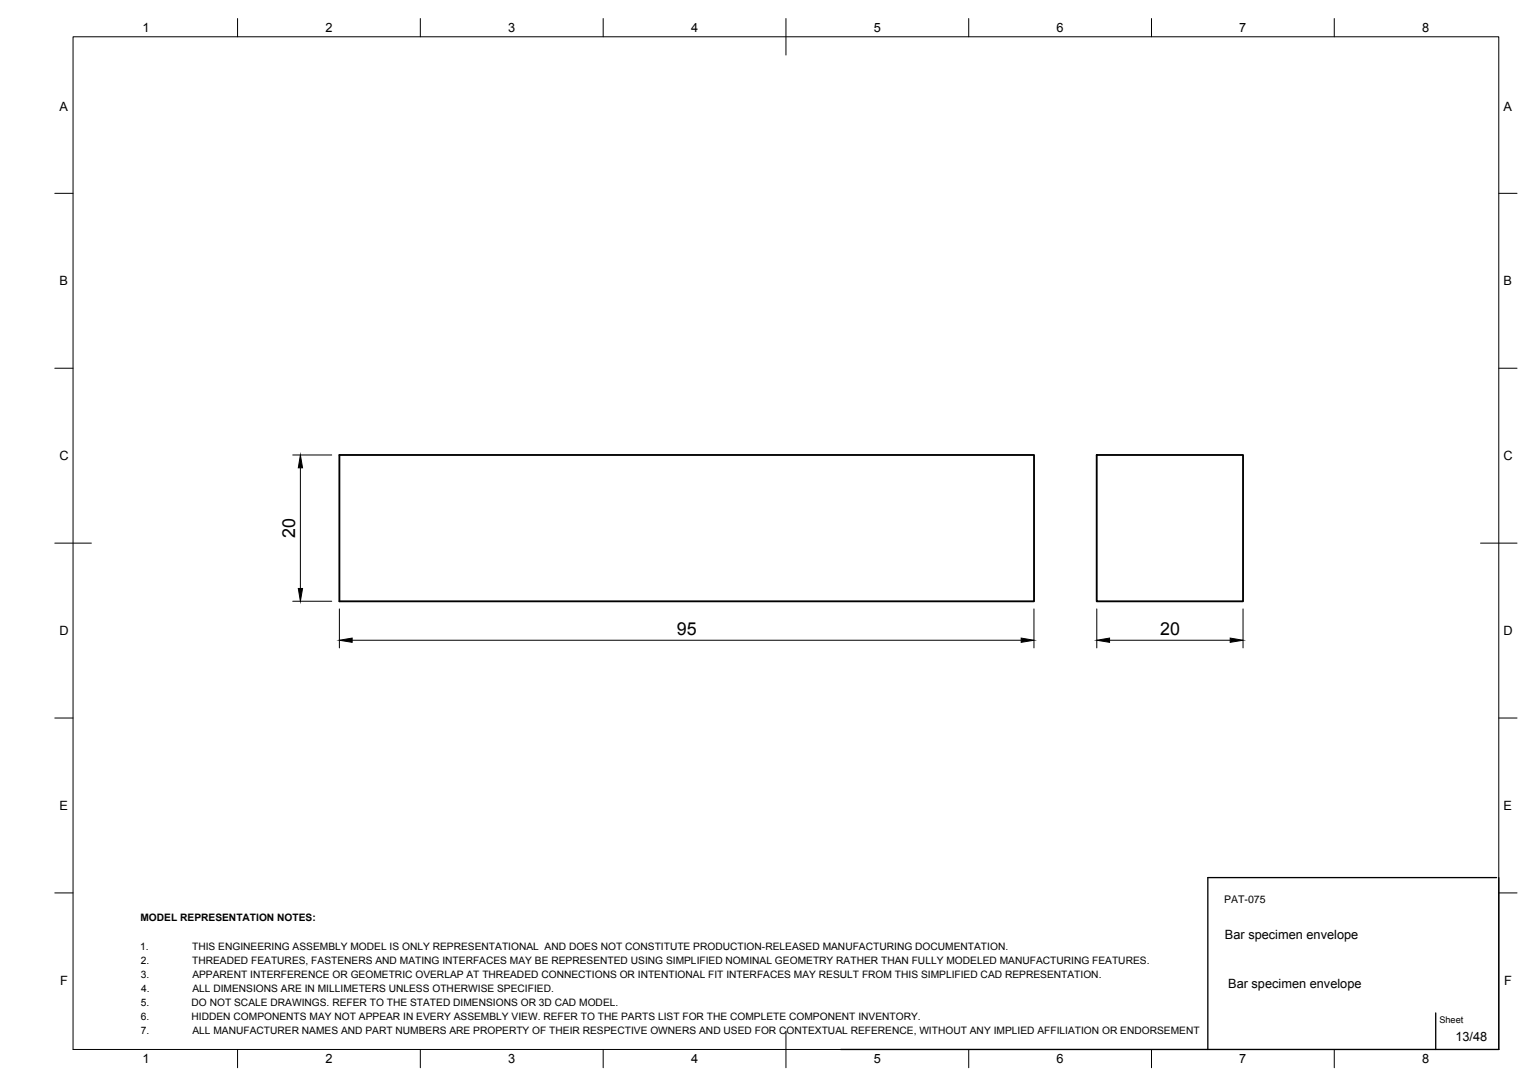
ISO-10303-21;
HEADER;
/* Generated by software containing ST-Developer
 * from STEP Tools, Inc. (www.steptools.com) 
 */

FILE_DESCRIPTION(
/* description */ ('Over-Centre Plunger Toggle Clamp on Slotted Fixture Frame'),
/* implementation_level */ '2;1');

FILE_NAME(
/* name */ 
'Bar specimen envelope.step',
/* time_stamp */ '2026-10-28T03:23:24-07:00',
/* author */ (''),
/* organization */ (''),
/* preprocessor_version */ 'ST-DEVELOPER v20.2',
/* originating_system */ 'Autodesk Translation Framework v15.17.0.0',
/* authorisation */ '');

FILE_SCHEMA (('AUTOMOTIVE_DESIGN { 1 0 10303 214 3 1 1 }'));
ENDSEC;

DATA;
#10=MECHANICAL_DESIGN_GEOMETRIC_PRESENTATION_REPRESENTATION('',(#521),#15212);
#437=SHAPE_REPRESENTATION_RELATIONSHIP('SRR','None',#15411,#479);
#479=ADVANCED_BREP_SHAPE_REPRESENTATION('',(#572),#15173);
#521=STYLED_ITEM('',(#15733),#572);
#572=MANIFOLD_SOLID_BREP('Body1',#8253);
#840=PLANE('',#9008);
#841=PLANE('',#9009);
#842=PLANE('',#9010);
#843=PLANE('',#9011);
#844=PLANE('',#9012);
#845=PLANE('',#9013);
#1203=FACE_OUTER_BOUND('',#1786,.T.);
#1204=FACE_OUTER_BOUND('',#1787,.T.);
#1205=FACE_OUTER_BOUND('',#1788,.T.);
#1206=FACE_OUTER_BOUND('',#1789,.T.);
#1207=FACE_OUTER_BOUND('',#1790,.T.);
#1208=FACE_OUTER_BOUND('',#1791,.T.);
#1786=EDGE_LOOP('',(#6091,#6092,#6093,#6094));
#1787=EDGE_LOOP('',(#6095,#6096,#6097,#6098));
#1788=EDGE_LOOP('',(#6099,#6100,#6101,#6102));
#1789=EDGE_LOOP('',(#6103,#6104,#6105,#6106));
#1790=EDGE_LOOP('',(#6107,#6108,#6109,#6110));
#1791=EDGE_LOOP('',(#6111,#6112,#6113,#6114));
#2374=LINE('',#12931,#3004);
#2375=LINE('',#12933,#3005);
#2376=LINE('',#12935,#3006);
#2377=LINE('',#12936,#3007);
#2378=LINE('',#12939,#3008);
#2379=LINE('',#12941,#3009);
#2380=LINE('',#12942,#3010);
#2381=LINE('',#12945,#3011);
#2382=LINE('',#12947,#3012);
#2383=LINE('',#12948,#3013);
#2384=LINE('',#12950,#3014);
#2385=LINE('',#12951,#3015);
#3004=VECTOR('',#10389,1.);
#3005=VECTOR('',#10390,1.);
#3006=VECTOR('',#10391,1.);
#3007=VECTOR('',#10392,1.);
#3008=VECTOR('',#10395,1.);
#3009=VECTOR('',#10396,1.);
#3010=VECTOR('',#10397,1.);
#3011=VECTOR('',#10400,1.);
#3012=VECTOR('',#10401,1.);
#3013=VECTOR('',#10402,1.);
#3014=VECTOR('',#10405,1.);
#3015=VECTOR('',#10406,1.);
#4033=VERTEX_POINT('',#12929);
#4034=VERTEX_POINT('',#12930);
#4035=VERTEX_POINT('',#12932);
#4036=VERTEX_POINT('',#12934);
#4037=VERTEX_POINT('',#12938);
#4038=VERTEX_POINT('',#12940);
#4039=VERTEX_POINT('',#12944);
#4040=VERTEX_POINT('',#12946);
#4806=EDGE_CURVE('',#4033,#4034,#2374,.T.);
#4807=EDGE_CURVE('',#4034,#4035,#2375,.T.);
#4808=EDGE_CURVE('',#4036,#4035,#2376,.T.);
#4809=EDGE_CURVE('',#4033,#4036,#2377,.T.);
#4810=EDGE_CURVE('',#4037,#4033,#2378,.T.);
#4811=EDGE_CURVE('',#4038,#4036,#2379,.T.);
#4812=EDGE_CURVE('',#4037,#4038,#2380,.T.);
#4813=EDGE_CURVE('',#4039,#4037,#2381,.T.);
#4814=EDGE_CURVE('',#4040,#4038,#2382,.T.);
#4815=EDGE_CURVE('',#4039,#4040,#2383,.T.);
#4816=EDGE_CURVE('',#4034,#4039,#2384,.T.);
#4817=EDGE_CURVE('',#4035,#4040,#2385,.T.);
#6091=ORIENTED_EDGE('',*,*,#4806,.T.);
#6092=ORIENTED_EDGE('',*,*,#4807,.T.);
#6093=ORIENTED_EDGE('',*,*,#4808,.F.);
#6094=ORIENTED_EDGE('',*,*,#4809,.F.);
#6095=ORIENTED_EDGE('',*,*,#4810,.T.);
#6096=ORIENTED_EDGE('',*,*,#4809,.T.);
#6097=ORIENTED_EDGE('',*,*,#4811,.F.);
#6098=ORIENTED_EDGE('',*,*,#4812,.F.);
#6099=ORIENTED_EDGE('',*,*,#4813,.T.);
#6100=ORIENTED_EDGE('',*,*,#4812,.T.);
#6101=ORIENTED_EDGE('',*,*,#4814,.F.);
#6102=ORIENTED_EDGE('',*,*,#4815,.F.);
#6103=ORIENTED_EDGE('',*,*,#4816,.T.);
#6104=ORIENTED_EDGE('',*,*,#4815,.T.);
#6105=ORIENTED_EDGE('',*,*,#4817,.F.);
#6106=ORIENTED_EDGE('',*,*,#4807,.F.);
#6107=ORIENTED_EDGE('',*,*,#4817,.T.);
#6108=ORIENTED_EDGE('',*,*,#4814,.T.);
#6109=ORIENTED_EDGE('',*,*,#4811,.T.);
#6110=ORIENTED_EDGE('',*,*,#4808,.T.);
#6111=ORIENTED_EDGE('',*,*,#4816,.F.);
#6112=ORIENTED_EDGE('',*,*,#4806,.F.);
#6113=ORIENTED_EDGE('',*,*,#4810,.F.);
#6114=ORIENTED_EDGE('',*,*,#4813,.F.);
#7875=ADVANCED_FACE('',(#1203),#840,.T.);
#7876=ADVANCED_FACE('',(#1204),#841,.T.);
#7877=ADVANCED_FACE('',(#1205),#842,.T.);
#7878=ADVANCED_FACE('',(#1206),#843,.T.);
#7879=ADVANCED_FACE('',(#1207),#844,.T.);
#7880=ADVANCED_FACE('',(#1208),#845,.F.);
#8253=CLOSED_SHELL('',(#7875,#7876,#7877,#7878,#7879,#7880));
#9007=AXIS2_PLACEMENT_3D('',#12927,#10385,#10386);
#9008=AXIS2_PLACEMENT_3D('',#12928,#10387,#10388);
#9009=AXIS2_PLACEMENT_3D('',#12937,#10393,#10394);
#9010=AXIS2_PLACEMENT_3D('',#12943,#10398,#10399);
#9011=AXIS2_PLACEMENT_3D('',#12949,#10403,#10404);
#9012=AXIS2_PLACEMENT_3D('',#12952,#10407,#10408);
#9013=AXIS2_PLACEMENT_3D('',#12953,#10409,#10410);
#10385=DIRECTION('axis',(0.,0.,1.));
#10386=DIRECTION('refdir',(1.,0.,0.));
#10387=DIRECTION('center_axis',(0.,1.,0.));
#10388=DIRECTION('ref_axis',(-1.,0.,0.));
#10389=DIRECTION('',(-1.,0.,0.));
#10390=DIRECTION('',(0.,0.,1.));
#10391=DIRECTION('',(-1.,0.,0.));
#10392=DIRECTION('',(0.,0.,1.));
#10393=DIRECTION('center_axis',(1.,0.,0.));
#10394=DIRECTION('ref_axis',(0.,1.,0.));
#10395=DIRECTION('',(0.,1.,0.));
#10396=DIRECTION('',(0.,1.,0.));
#10397=DIRECTION('',(0.,0.,1.));
#10398=DIRECTION('center_axis',(0.,-1.,0.));
#10399=DIRECTION('ref_axis',(1.,0.,0.));
#10400=DIRECTION('',(1.,0.,0.));
#10401=DIRECTION('',(1.,0.,0.));
#10402=DIRECTION('',(0.,0.,1.));
#10403=DIRECTION('center_axis',(-1.,0.,0.));
#10404=DIRECTION('ref_axis',(0.,-1.,0.));
#10405=DIRECTION('',(0.,-1.,0.));
#10406=DIRECTION('',(0.,-1.,0.));
#10407=DIRECTION('center_axis',(0.,0.,1.));
#10408=DIRECTION('ref_axis',(1.,0.,0.));
#10409=DIRECTION('center_axis',(0.,0.,1.));
#10410=DIRECTION('ref_axis',(1.,0.,0.));
#12927=CARTESIAN_POINT('',(0.,0.,0.));
#12928=CARTESIAN_POINT('Origin',(1.,3.5,1.));
#12929=CARTESIAN_POINT('',(1.,3.5,1.));
#12930=CARTESIAN_POINT('',(-1.,3.5,1.));
#12931=CARTESIAN_POINT('',(1.,3.5,1.));
#12932=CARTESIAN_POINT('',(-1.,3.5,3.));
#12933=CARTESIAN_POINT('',(-1.,3.5,1.));
#12934=CARTESIAN_POINT('',(1.,3.5,3.));
#12935=CARTESIAN_POINT('',(1.,3.5,3.));
#12936=CARTESIAN_POINT('',(1.,3.5,1.));
#12937=CARTESIAN_POINT('Origin',(1.,-6.,1.));
#12938=CARTESIAN_POINT('',(1.,-6.,1.));
#12939=CARTESIAN_POINT('',(1.,-6.,1.));
#12940=CARTESIAN_POINT('',(1.,-6.,3.));
#12941=CARTESIAN_POINT('',(1.,-6.,3.));
#12942=CARTESIAN_POINT('',(1.,-6.,1.));
#12943=CARTESIAN_POINT('Origin',(-1.,-6.,1.));
#12944=CARTESIAN_POINT('',(-1.,-6.,1.));
#12945=CARTESIAN_POINT('',(-1.,-6.,1.));
#12946=CARTESIAN_POINT('',(-1.,-6.,3.));
#12947=CARTESIAN_POINT('',(-1.,-6.,3.));
#12948=CARTESIAN_POINT('',(-1.,-6.,1.));
#12949=CARTESIAN_POINT('Origin',(-1.,3.5,1.));
#12950=CARTESIAN_POINT('',(-1.,3.5,1.));
#12951=CARTESIAN_POINT('',(-1.,3.5,3.));
#12952=CARTESIAN_POINT('Origin',(0.,-1.25,3.));
#12953=CARTESIAN_POINT('Origin',(0.,-1.25,1.));
#15123=UNCERTAINTY_MEASURE_WITH_UNIT(LENGTH_MEASURE(0.001),#15213,
'DISTANCE_ACCURACY_VALUE',
'Maximum model space distance between geometric entities at asserted c
onnectivities');
#15162=UNCERTAINTY_MEASURE_WITH_UNIT(LENGTH_MEASURE(0.001),#15213,
'DISTANCE_ACCURACY_VALUE',
'Maximum model space distance between geometric entities at asserted c
onnectivities');
#15173=(
GEOMETRIC_REPRESENTATION_CONTEXT(3)
GLOBAL_UNCERTAINTY_ASSIGNED_CONTEXT((#15123))
GLOBAL_UNIT_ASSIGNED_CONTEXT((#15213,#15215,#15216))
REPRESENTATION_CONTEXT('','3D')
);
#15212=(
GEOMETRIC_REPRESENTATION_CONTEXT(3)
GLOBAL_UNCERTAINTY_ASSIGNED_CONTEXT((#15162))
GLOBAL_UNIT_ASSIGNED_CONTEXT((#15213,#15215,#15216))
REPRESENTATION_CONTEXT('','3D')
);
#15213=(
LENGTH_UNIT()
NAMED_UNIT(*)
SI_UNIT(.CENTI.,.METRE.)
);
#15215=(
NAMED_UNIT(*)
PLANE_ANGLE_UNIT()
SI_UNIT($,.RADIAN.)
);
#15216=(
NAMED_UNIT(*)
SI_UNIT($,.STERADIAN.)
SOLID_ANGLE_UNIT()
);
#15227=SHAPE_DEFINITION_REPRESENTATION(#15276,#15411);
#15276=PRODUCT_DEFINITION_SHAPE('',$,#15461);
#15411=SHAPE_REPRESENTATION('',(#9007),#15173);
#15450=PRODUCT_DEFINITION_CONTEXT('part definition',#15599,'design');
#15461=PRODUCT_DEFINITION('Bar specimen envelope',
'Bar specimen envelope',#15510,#15450);
#15510=PRODUCT_DEFINITION_FORMATION('',$,#15611);
#15599=APPLICATION_CONTEXT(
'Core Data for Automotive Mechanical Design Process');
#15600=PRODUCT_CONTEXT('part definition',#15599,'mechanical');
#15611=PRODUCT('Bar specimen envelope','Bar specimen envelope',
'Bar specimen envelope',(#15600));
#15727=COLOUR_RGB('Off White',0.89,0.88,0.83);
#15728=FILL_AREA_STYLE_COLOUR('',#15727);
#15729=FILL_AREA_STYLE('',(#15728));
#15730=SURFACE_STYLE_FILL_AREA(#15729);
#15731=SURFACE_SIDE_STYLE('',(#15730));
#15732=SURFACE_STYLE_USAGE(.BOTH.,#15731);
#15733=PRESENTATION_STYLE_ASSIGNMENT((#15732));
ENDSEC;
END-ISO-10303-21;
